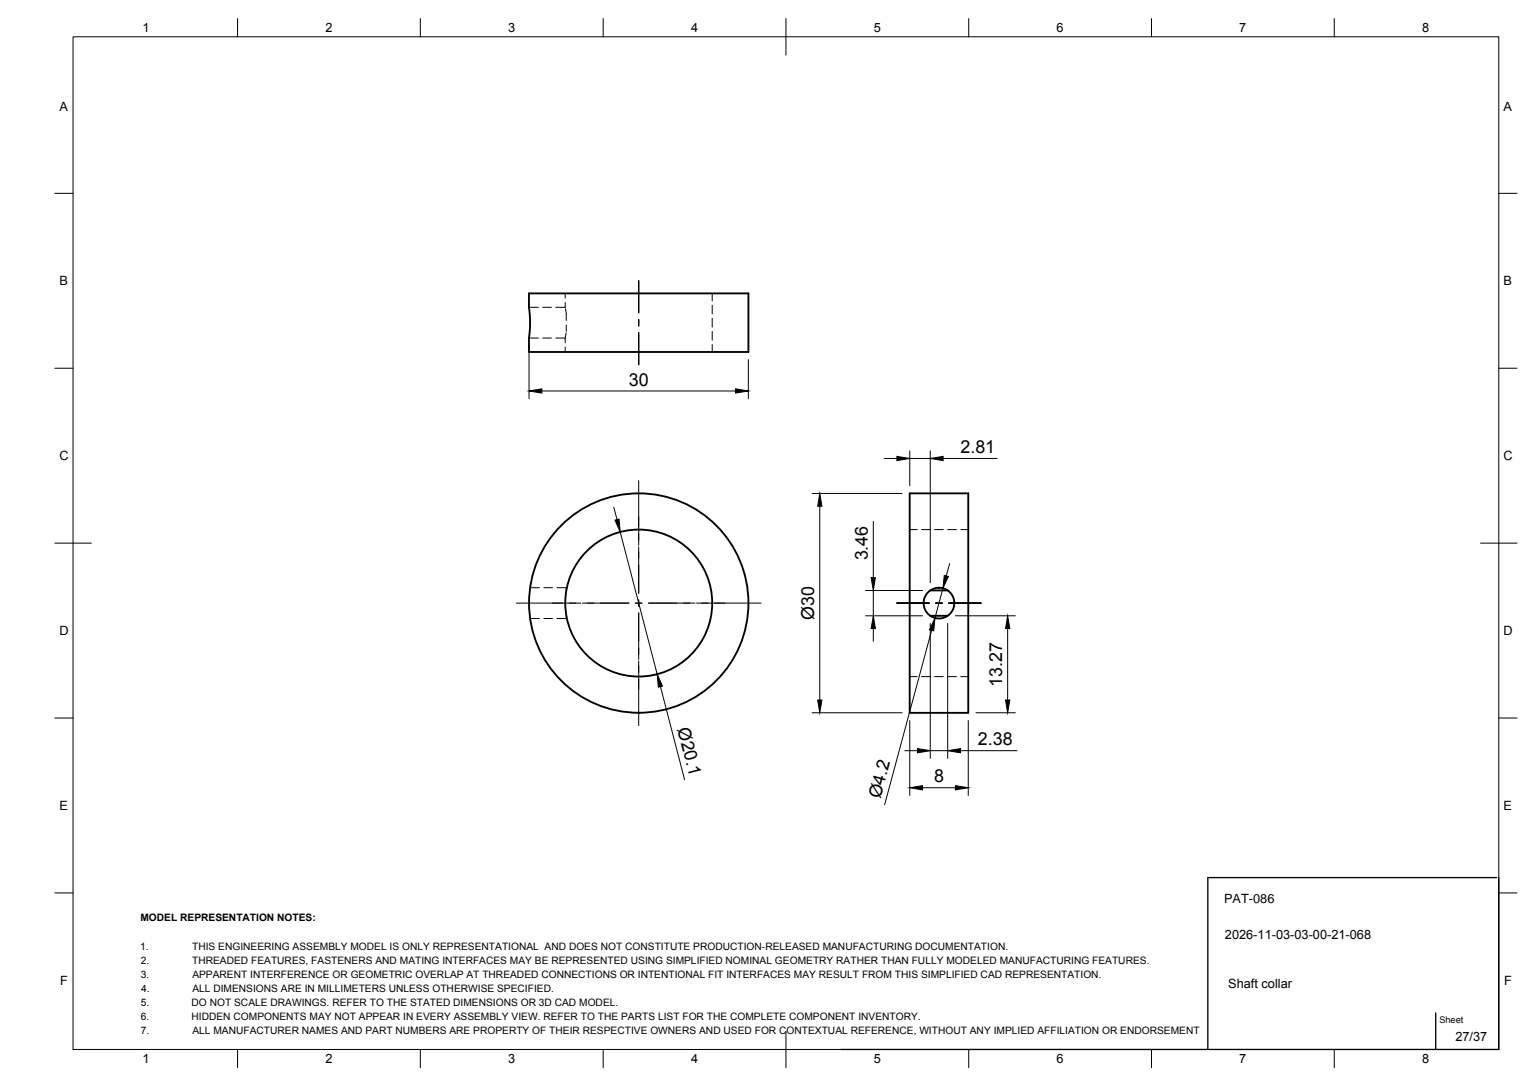
ISO-10303-21;
HEADER;
/* Generated by software containing ST-Developer
 * from STEP Tools, Inc. (www.steptools.com) 
 */

FILE_DESCRIPTION(
/* description */ ('Ratchet and pawl hand winch drum'),
/* implementation_level */ '2;1');

FILE_NAME(
/* name */ 'Shaft collar.step',
/* time_stamp */ '2026-10-27T12:42:58-07:00',
/* author */ (''),
/* organization */ (''),
/* preprocessor_version */ 'ST-DEVELOPER v20.2',
/* originating_system */ 'Autodesk Translation Framework v15.17.0.0',
/* authorisation */ '');

FILE_SCHEMA (('AUTOMOTIVE_DESIGN { 1 0 10303 214 3 1 1 }'));
ENDSEC;

DATA;
#10=MECHANICAL_DESIGN_GEOMETRIC_PRESENTATION_REPRESENTATION('',(#411),#11801);
#297=B_SPLINE_CURVE_WITH_KNOTS('',3,(#10598,#10599,#10600,#10601,#10602,
#10603,#10604,#10605,#10606,#10607,#10608,#10609,#10610,#10611),
 .UNSPECIFIED.,.F.,.F.,(4,2,2,2,2,2,4),(0.75600573798702,0.793568827564647,
0.872922520054201,0.952276212543756,1.03162990503331,1.11098359752287,1.14854668710049),
 .UNSPECIFIED.);
#298=B_SPLINE_CURVE_WITH_KNOTS('',3,(#10617,#10618,#10619,#10620,#10621,
#10622,#10623,#10624,#10625,#10626,#10627,#10628,#10629,#10630,#10631,#10632,
#10633,#10634),.UNSPECIFIED.,.F.,.F.,(4,2,2,2,2,2,2,2,4),(0.,0.079216580773363,
0.158433161546726,0.23764869707457,0.316864232602414,0.396079768130259,
0.475295303658103,0.554511884431466,0.633728465204829),.UNSPECIFIED.);
#299=B_SPLINE_CURVE_WITH_KNOTS('',3,(#10635,#10636,#10637,#10638,#10639,
#10640,#10641,#10642,#10643,#10644,#10645,#10646,#10647,#10648,#10649,#10650,
#10651,#10652),.UNSPECIFIED.,.F.,.F.,(4,2,2,2,2,2,2,2,4),(0.633728465204829,
0.712945045978192,0.792161626751555,0.871377162279399,0.950592697807243,
1.02980823333509,1.10902376886293,1.18824034963629,1.26745693040966),
 .UNSPECIFIED.);
#300=B_SPLINE_CURVE_WITH_KNOTS('',3,(#10655,#10656,#10657,#10658,#10659,
#10660,#10661,#10662,#10663,#10664,#10665,#10666,#10667,#10668),
 .UNSPECIFIED.,.F.,.F.,(4,2,2,2,2,2,4),(0.121154929624515,0.158718019202143,
0.238071711691697,0.317425404181252,0.396779096670807,0.476132789160362,
0.513695878737989),.UNSPECIFIED.);
#342=SHAPE_REPRESENTATION_RELATIONSHIP('SRR','None',#11970,#376);
#376=ADVANCED_BREP_SHAPE_REPRESENTATION('',(#444),#11787);
#411=STYLED_ITEM('',(#12213),#444);
#444=MANIFOLD_SOLID_BREP('Body1',#6290);
#564=FACE_BOUND('',#1514,.T.);
#565=FACE_BOUND('',#1516,.T.);
#566=FACE_BOUND('',#1518,.T.);
#567=FACE_BOUND('',#1520,.T.);
#728=PLANE('',#7057);
#729=PLANE('',#7062);
#730=PLANE('',#7069);
#731=PLANE('',#7070);
#1046=FACE_OUTER_BOUND('',#1510,.T.);
#1047=FACE_OUTER_BOUND('',#1511,.T.);
#1048=FACE_OUTER_BOUND('',#1512,.T.);
#1049=FACE_OUTER_BOUND('',#1513,.T.);
#1050=FACE_OUTER_BOUND('',#1515,.T.);
#1051=FACE_OUTER_BOUND('',#1517,.T.);
#1052=FACE_OUTER_BOUND('',#1519,.T.);
#1510=EDGE_LOOP('',(#5107,#5108));
#1511=EDGE_LOOP('',(#5109,#5110,#5111,#5112,#5113,#5114,#5115,#5116,#5117));
#1512=EDGE_LOOP('',(#5118,#5119,#5120));
#1513=EDGE_LOOP('',(#5121,#5122,#5123,#5124));
#1514=EDGE_LOOP('',(#5125,#5126,#5127,#5128));
#1515=EDGE_LOOP('',(#5129,#5130,#5131,#5132));
#1516=EDGE_LOOP('',(#5133,#5134));
#1517=EDGE_LOOP('',(#5135));
#1518=EDGE_LOOP('',(#5136));
#1519=EDGE_LOOP('',(#5137));
#1520=EDGE_LOOP('',(#5138));
#1959=LINE('',#10594,#2470);
#1960=LINE('',#10615,#2471);
#1961=LINE('',#10670,#2472);
#1962=LINE('',#10675,#2473);
#1963=LINE('',#10681,#2474);
#2470=VECTOR('',#8378,1.);
#2471=VECTOR('',#8385,0.21);
#2472=VECTOR('',#8390,1.);
#2473=VECTOR('',#8395,1.005);
#2474=VECTOR('',#8402,1.5);
#2863=CIRCLE('',#7058,0.21);
#2864=CIRCLE('',#7060,0.21);
#2865=CIRCLE('',#7061,0.21);
#2866=CIRCLE('',#7064,1.005);
#2867=CIRCLE('',#7065,1.005);
#2868=CIRCLE('',#7067,1.5);
#2869=CIRCLE('',#7068,1.5);
#3234=VERTEX_POINT('',#10592);
#3235=VERTEX_POINT('',#10593);
#3236=VERTEX_POINT('',#10597);
#3237=VERTEX_POINT('',#10612);
#3238=VERTEX_POINT('',#10614);
#3239=VERTEX_POINT('',#10616);
#3240=VERTEX_POINT('',#10653);
#3241=VERTEX_POINT('',#10672);
#3242=VERTEX_POINT('',#10674);
#3243=VERTEX_POINT('',#10678);
#3244=VERTEX_POINT('',#10680);
#3897=EDGE_CURVE('',#3234,#3235,#1959,.T.);
#3898=EDGE_CURVE('',#3234,#3235,#2863,.T.);
#3899=EDGE_CURVE('',#3236,#3234,#297,.T.);
#3900=EDGE_CURVE('',#3237,#3236,#2864,.T.);
#3901=EDGE_CURVE('',#3237,#3238,#1960,.T.);
#3902=EDGE_CURVE('',#3239,#3238,#298,.T.);
#3903=EDGE_CURVE('',#3238,#3239,#299,.T.);
#3904=EDGE_CURVE('',#3240,#3237,#2865,.T.);
#3905=EDGE_CURVE('',#3235,#3240,#300,.T.);
#3906=EDGE_CURVE('',#3240,#3236,#1961,.T.);
#3907=EDGE_CURVE('',#3241,#3241,#2866,.T.);
#3908=EDGE_CURVE('',#3241,#3242,#1962,.T.);
#3909=EDGE_CURVE('',#3242,#3242,#2867,.T.);
#3910=EDGE_CURVE('',#3243,#3243,#2868,.T.);
#3911=EDGE_CURVE('',#3243,#3244,#1963,.T.);
#3912=EDGE_CURVE('',#3244,#3244,#2869,.T.);
#5107=ORIENTED_EDGE('',*,*,#3897,.F.);
#5108=ORIENTED_EDGE('',*,*,#3898,.T.);
#5109=ORIENTED_EDGE('',*,*,#3899,.F.);
#5110=ORIENTED_EDGE('',*,*,#3900,.F.);
#5111=ORIENTED_EDGE('',*,*,#3901,.T.);
#5112=ORIENTED_EDGE('',*,*,#3902,.F.);
#5113=ORIENTED_EDGE('',*,*,#3903,.F.);
#5114=ORIENTED_EDGE('',*,*,#3901,.F.);
#5115=ORIENTED_EDGE('',*,*,#3904,.F.);
#5116=ORIENTED_EDGE('',*,*,#3905,.F.);
#5117=ORIENTED_EDGE('',*,*,#3898,.F.);
#5118=ORIENTED_EDGE('',*,*,#3906,.F.);
#5119=ORIENTED_EDGE('',*,*,#3904,.T.);
#5120=ORIENTED_EDGE('',*,*,#3900,.T.);
#5121=ORIENTED_EDGE('',*,*,#3907,.F.);
#5122=ORIENTED_EDGE('',*,*,#3908,.T.);
#5123=ORIENTED_EDGE('',*,*,#3909,.T.);
#5124=ORIENTED_EDGE('',*,*,#3908,.F.);
#5125=ORIENTED_EDGE('',*,*,#3905,.T.);
#5126=ORIENTED_EDGE('',*,*,#3906,.T.);
#5127=ORIENTED_EDGE('',*,*,#3899,.T.);
#5128=ORIENTED_EDGE('',*,*,#3897,.T.);
#5129=ORIENTED_EDGE('',*,*,#3910,.F.);
#5130=ORIENTED_EDGE('',*,*,#3911,.T.);
#5131=ORIENTED_EDGE('',*,*,#3912,.T.);
#5132=ORIENTED_EDGE('',*,*,#3911,.F.);
#5133=ORIENTED_EDGE('',*,*,#3902,.T.);
#5134=ORIENTED_EDGE('',*,*,#3903,.T.);
#5135=ORIENTED_EDGE('',*,*,#3910,.T.);
#5136=ORIENTED_EDGE('',*,*,#3907,.T.);
#5137=ORIENTED_EDGE('',*,*,#3912,.F.);
#5138=ORIENTED_EDGE('',*,*,#3909,.F.);
#5878=CYLINDRICAL_SURFACE('',#7059,0.21);
#5879=CYLINDRICAL_SURFACE('',#7063,1.005);
#5880=CYLINDRICAL_SURFACE('',#7066,1.5);
#6116=ADVANCED_FACE('',(#1046),#728,.T.);
#6117=ADVANCED_FACE('',(#1047),#5878,.F.);
#6118=ADVANCED_FACE('',(#1048),#729,.T.);
#6119=ADVANCED_FACE('',(#1049,#564),#5879,.F.);
#6120=ADVANCED_FACE('',(#1050,#565),#5880,.T.);
#6121=ADVANCED_FACE('',(#1051,#566),#730,.T.);
#6122=ADVANCED_FACE('',(#1052,#567),#731,.F.);
#6290=CLOSED_SHELL('',(#6116,#6117,#6118,#6119,#6120,#6121,#6122));
#7056=AXIS2_PLACEMENT_3D('',#10590,#8374,#8375);
#7057=AXIS2_PLACEMENT_3D('',#10591,#8376,#8377);
#7058=AXIS2_PLACEMENT_3D('',#10595,#8379,#8380);
#7059=AXIS2_PLACEMENT_3D('',#10596,#8381,#8382);
#7060=AXIS2_PLACEMENT_3D('',#10613,#8383,#8384);
#7061=AXIS2_PLACEMENT_3D('',#10654,#8386,#8387);
#7062=AXIS2_PLACEMENT_3D('',#10669,#8388,#8389);
#7063=AXIS2_PLACEMENT_3D('',#10671,#8391,#8392);
#7064=AXIS2_PLACEMENT_3D('',#10673,#8393,#8394);
#7065=AXIS2_PLACEMENT_3D('',#10676,#8396,#8397);
#7066=AXIS2_PLACEMENT_3D('',#10677,#8398,#8399);
#7067=AXIS2_PLACEMENT_3D('',#10679,#8400,#8401);
#7068=AXIS2_PLACEMENT_3D('',#10682,#8403,#8404);
#7069=AXIS2_PLACEMENT_3D('',#10683,#8405,#8406);
#7070=AXIS2_PLACEMENT_3D('',#10684,#8407,#8408);
#8374=DIRECTION('axis',(0.,0.,1.));
#8375=DIRECTION('refdir',(1.,0.,0.));
#8376=DIRECTION('center_axis',(0.,0.,1.));
#8377=DIRECTION('ref_axis',(1.,0.,0.));
#8378=DIRECTION('',(0.,1.,0.));
#8379=DIRECTION('center_axis',(0.,0.,1.));
#8380=DIRECTION('ref_axis',(1.,0.,0.));
#8381=DIRECTION('center_axis',(0.,0.,1.));
#8382=DIRECTION('ref_axis',(1.,0.,0.));
#8383=DIRECTION('center_axis',(0.,0.,1.));
#8384=DIRECTION('ref_axis',(1.,0.,0.));
#8385=DIRECTION('',(0.,0.,1.));
#8386=DIRECTION('center_axis',(0.,0.,1.));
#8387=DIRECTION('ref_axis',(1.,0.,0.));
#8388=DIRECTION('center_axis',(0.,0.,1.));
#8389=DIRECTION('ref_axis',(1.,0.,0.));
#8390=DIRECTION('',(0.,-1.,0.));
#8391=DIRECTION('center_axis',(0.,1.,0.));
#8392=DIRECTION('ref_axis',(1.,0.,0.));
#8393=DIRECTION('center_axis',(0.,-1.,0.));
#8394=DIRECTION('ref_axis',(1.,0.,0.));
#8395=DIRECTION('',(0.,-1.,0.));
#8396=DIRECTION('center_axis',(0.,-1.,0.));
#8397=DIRECTION('ref_axis',(1.,0.,0.));
#8398=DIRECTION('center_axis',(0.,1.,0.));
#8399=DIRECTION('ref_axis',(1.,0.,0.));
#8400=DIRECTION('center_axis',(0.,1.,0.));
#8401=DIRECTION('ref_axis',(1.,0.,0.));
#8402=DIRECTION('',(0.,-1.,0.));
#8403=DIRECTION('center_axis',(0.,1.,0.));
#8404=DIRECTION('ref_axis',(1.,0.,0.));
#8405=DIRECTION('center_axis',(0.,1.,0.));
#8406=DIRECTION('ref_axis',(1.,0.,0.));
#8407=DIRECTION('center_axis',(0.,1.,0.));
#8408=DIRECTION('ref_axis',(1.,0.,0.));
#10590=CARTESIAN_POINT('',(0.,0.,0.));
#10591=CARTESIAN_POINT('Origin',(0.,-1.25,7.52));
#10592=CARTESIAN_POINT('',(0.172988438920056,-1.36905880899792,7.52));
#10593=CARTESIAN_POINT('',(0.172988438920056,-1.13094119100209,7.52));
#10594=CARTESIAN_POINT('',(0.172988438920056,-1.65,7.52));
#10595=CARTESIAN_POINT('Origin',(0.,-1.25,7.52));
#10596=CARTESIAN_POINT('Origin',(0.,-1.25,7.52));
#10597=CARTESIAN_POINT('',(-0.172988438920056,-1.36905880899792,7.52));
#10598=CARTESIAN_POINT('Ctrl Pts',(-0.172988438920056,-1.36905880899792,
7.52));
#10599=CARTESIAN_POINT('Ctrl Pts',(-0.165594865311314,-1.37980142239529,
7.52129192197638));
#10600=CARTESIAN_POINT('Ctrl Pts',(-0.157297138725606,-1.38968770937274,
7.52265394943905));
#10601=CARTESIAN_POINT('Ctrl Pts',(-0.129892073845076,-1.41709277425327,
7.5267480843909));
#10602=CARTESIAN_POINT('Ctrl Pts',(-0.106330167759284,-1.43324205633295,
7.52969589327638));
#10603=CARTESIAN_POINT('Ctrl Pts',(-0.0546129046324105,-1.45469779396491,
7.53385029472357));
#10604=CARTESIAN_POINT('Ctrl Pts',(-0.0264512308298517,-1.46,7.535));
#10605=CARTESIAN_POINT('Ctrl Pts',(0.0264512308298516,-1.46,7.535));
#10606=CARTESIAN_POINT('Ctrl Pts',(0.0546129046324104,-1.45469779396491,
7.53385029472357));
#10607=CARTESIAN_POINT('Ctrl Pts',(0.106330167759284,-1.43324205633295,
7.52969589327638));
#10608=CARTESIAN_POINT('Ctrl Pts',(0.129892073845076,-1.41709277425327,
7.5267480843909));
#10609=CARTESIAN_POINT('Ctrl Pts',(0.157297138725606,-1.38968770937274,
7.52265394943905));
#10610=CARTESIAN_POINT('Ctrl Pts',(0.165594865311315,-1.37980142239529,
7.52129192197638));
#10611=CARTESIAN_POINT('Ctrl Pts',(0.172988438920056,-1.36905880899792,
7.52));
#10612=CARTESIAN_POINT('',(-0.21,-1.25,7.52));
#10613=CARTESIAN_POINT('Origin',(0.,-1.25,7.52));
#10614=CARTESIAN_POINT('',(-0.21,-1.25,8.01522725533839));
#10615=CARTESIAN_POINT('',(-0.21,-1.25,7.52));
#10616=CARTESIAN_POINT('',(0.21,-1.25,8.01522725533839));
#10617=CARTESIAN_POINT('Ctrl Pts',(0.21,-1.25,8.01522725533839));
#10618=CARTESIAN_POINT('Ctrl Pts',(0.21,-1.27640552692445,8.01522725533839));
#10619=CARTESIAN_POINT('Ctrl Pts',(0.204715737269596,-1.30454707409071,
8.01600415954412));
#10620=CARTESIAN_POINT('Ctrl Pts',(0.183273763036332,-1.35627626890513,
8.01880073282317));
#10621=CARTESIAN_POINT('Ctrl Pts',(0.167117923970394,-1.37986692412796,
8.02077897157582));
#10622=CARTESIAN_POINT('Ctrl Pts',(0.129867169887369,-1.41711767821098,
8.02448481141327));
#10623=CARTESIAN_POINT('Ctrl Pts',(0.106276408305765,-1.43327371000135,
8.02645455657129));
#10624=CARTESIAN_POINT('Ctrl Pts',(0.0545468514059001,-1.45471582482622,
8.02923165515645));
#10625=CARTESIAN_POINT('Ctrl Pts',(0.0264051785092814,-1.46,8.03));
#10626=CARTESIAN_POINT('Ctrl Pts',(-0.0264051785092814,-1.46,8.03));
#10627=CARTESIAN_POINT('Ctrl Pts',(-0.0545468514059,-1.45471582482622,8.02923165515645));
#10628=CARTESIAN_POINT('Ctrl Pts',(-0.106276408305765,-1.43327371000135,
8.02645455657129));
#10629=CARTESIAN_POINT('Ctrl Pts',(-0.129867169887369,-1.41711767821098,
8.02448481141327));
#10630=CARTESIAN_POINT('Ctrl Pts',(-0.167117923970394,-1.37986692412796,
8.02077897157582));
#10631=CARTESIAN_POINT('Ctrl Pts',(-0.183273763036331,-1.35627626890513,
8.01880073282317));
#10632=CARTESIAN_POINT('Ctrl Pts',(-0.204715737269596,-1.30454707409071,
8.01600415954412));
#10633=CARTESIAN_POINT('Ctrl Pts',(-0.21,-1.27640552692445,8.01522725533839));
#10634=CARTESIAN_POINT('Ctrl Pts',(-0.21,-1.25,8.01522725533839));
#10635=CARTESIAN_POINT('Ctrl Pts',(-0.21,-1.25,8.01522725533839));
#10636=CARTESIAN_POINT('Ctrl Pts',(-0.21,-1.22359447307555,8.01522725533839));
#10637=CARTESIAN_POINT('Ctrl Pts',(-0.204715737269596,-1.19545292590929,
8.01600415954412));
#10638=CARTESIAN_POINT('Ctrl Pts',(-0.183273763036332,-1.14372373109487,
8.01880073282317));
#10639=CARTESIAN_POINT('Ctrl Pts',(-0.167117923970394,-1.12013307587204,
8.02077897157582));
#10640=CARTESIAN_POINT('Ctrl Pts',(-0.129867169887369,-1.08288232178902,
8.02448481141327));
#10641=CARTESIAN_POINT('Ctrl Pts',(-0.106276408305765,-1.06672628999865,
8.02645455657129));
#10642=CARTESIAN_POINT('Ctrl Pts',(-0.0545468514059001,-1.04528417517378,
8.02923165515645));
#10643=CARTESIAN_POINT('Ctrl Pts',(-0.0264051785092814,-1.04,8.03));
#10644=CARTESIAN_POINT('Ctrl Pts',(0.0264051785092814,-1.04,8.03));
#10645=CARTESIAN_POINT('Ctrl Pts',(0.0545468514059002,-1.04528417517378,
8.02923165515645));
#10646=CARTESIAN_POINT('Ctrl Pts',(0.106276408305765,-1.06672628999865,
8.02645455657129));
#10647=CARTESIAN_POINT('Ctrl Pts',(0.129867169887369,-1.08288232178902,
8.02448481141327));
#10648=CARTESIAN_POINT('Ctrl Pts',(0.167117923970394,-1.12013307587204,
8.02077897157582));
#10649=CARTESIAN_POINT('Ctrl Pts',(0.183273763036331,-1.14372373109487,
8.01880073282317));
#10650=CARTESIAN_POINT('Ctrl Pts',(0.204715737269596,-1.19545292590929,
8.01600415954412));
#10651=CARTESIAN_POINT('Ctrl Pts',(0.21,-1.22359447307555,8.01522725533839));
#10652=CARTESIAN_POINT('Ctrl Pts',(0.21,-1.25,8.01522725533839));
#10653=CARTESIAN_POINT('',(-0.172988438920056,-1.13094119100209,7.52));
#10654=CARTESIAN_POINT('Origin',(0.,-1.25,7.52));
#10655=CARTESIAN_POINT('Ctrl Pts',(0.172988438920056,-1.13094119100209,
7.52));
#10656=CARTESIAN_POINT('Ctrl Pts',(0.165594865311315,-1.12019857760471,
7.52129192197638));
#10657=CARTESIAN_POINT('Ctrl Pts',(0.157297138725606,-1.11031229062726,
7.52265394943905));
#10658=CARTESIAN_POINT('Ctrl Pts',(0.129892073845076,-1.08290722574673,
7.5267480843909));
#10659=CARTESIAN_POINT('Ctrl Pts',(0.106330167759284,-1.06675794366705,
7.52969589327638));
#10660=CARTESIAN_POINT('Ctrl Pts',(0.0546129046324104,-1.04530220603509,
7.53385029472357));
#10661=CARTESIAN_POINT('Ctrl Pts',(0.0264512308298516,-1.04,7.535));
#10662=CARTESIAN_POINT('Ctrl Pts',(-0.0264512308298516,-1.04,7.535));
#10663=CARTESIAN_POINT('Ctrl Pts',(-0.0546129046324104,-1.04530220603509,
7.53385029472357));
#10664=CARTESIAN_POINT('Ctrl Pts',(-0.106330167759284,-1.06675794366705,
7.52969589327638));
#10665=CARTESIAN_POINT('Ctrl Pts',(-0.129892073845076,-1.08290722574673,
7.5267480843909));
#10666=CARTESIAN_POINT('Ctrl Pts',(-0.157297138725606,-1.11031229062726,
7.52265394943905));
#10667=CARTESIAN_POINT('Ctrl Pts',(-0.165594865311315,-1.12019857760471,
7.52129192197638));
#10668=CARTESIAN_POINT('Ctrl Pts',(-0.172988438920056,-1.13094119100209,
7.52));
#10669=CARTESIAN_POINT('Origin',(0.,-1.25,7.52));
#10670=CARTESIAN_POINT('',(-0.172988438920056,-1.65,7.52));
#10671=CARTESIAN_POINT('Origin',(0.,-1.65,6.53));
#10672=CARTESIAN_POINT('',(-1.005,-0.85,6.53));
#10673=CARTESIAN_POINT('Origin',(0.,-0.85,6.53));
#10674=CARTESIAN_POINT('',(-1.005,-1.65,6.53));
#10675=CARTESIAN_POINT('',(-1.005,-1.65,6.53));
#10676=CARTESIAN_POINT('Origin',(0.,-1.65,6.53));
#10677=CARTESIAN_POINT('Origin',(0.,-1.65,6.53));
#10678=CARTESIAN_POINT('',(-1.5,-0.85,6.53));
#10679=CARTESIAN_POINT('Origin',(0.,-0.85,6.53));
#10680=CARTESIAN_POINT('',(-1.5,-1.65,6.53));
#10681=CARTESIAN_POINT('',(-1.5,-1.65,6.53));
#10682=CARTESIAN_POINT('Origin',(0.,-1.65,6.53));
#10683=CARTESIAN_POINT('Origin',(0.,-0.85,6.53));
#10684=CARTESIAN_POINT('Origin',(0.,-1.65,6.53));
#11747=UNCERTAINTY_MEASURE_WITH_UNIT(LENGTH_MEASURE(0.001),#11802,
'DISTANCE_ACCURACY_VALUE',
'Maximum model space distance between geometric entities at asserted c
onnectivities');
#11761=UNCERTAINTY_MEASURE_WITH_UNIT(LENGTH_MEASURE(0.001),#11802,
'DISTANCE_ACCURACY_VALUE',
'Maximum model space distance between geometric entities at asserted c
onnectivities');
#11787=(
GEOMETRIC_REPRESENTATION_CONTEXT(3)
GLOBAL_UNCERTAINTY_ASSIGNED_CONTEXT((#11747))
GLOBAL_UNIT_ASSIGNED_CONTEXT((#11802,#11804,#11805))
REPRESENTATION_CONTEXT('','3D')
);
#11801=(
GEOMETRIC_REPRESENTATION_CONTEXT(3)
GLOBAL_UNCERTAINTY_ASSIGNED_CONTEXT((#11761))
GLOBAL_UNIT_ASSIGNED_CONTEXT((#11802,#11804,#11805))
REPRESENTATION_CONTEXT('','3D')
);
#11802=(
LENGTH_UNIT()
NAMED_UNIT(*)
SI_UNIT(.CENTI.,.METRE.)
);
#11804=(
NAMED_UNIT(*)
PLANE_ANGLE_UNIT()
SI_UNIT($,.RADIAN.)
);
#11805=(
NAMED_UNIT(*)
SI_UNIT($,.STERADIAN.)
SOLID_ANGLE_UNIT()
);
#11831=SHAPE_DEFINITION_REPRESENTATION(#11872,#11970);
#11872=PRODUCT_DEFINITION_SHAPE('',$,#12010);
#11970=SHAPE_REPRESENTATION('',(#7056),#11787);
#11984=PRODUCT_DEFINITION_CONTEXT('part definition',#12103,'design');
#12010=PRODUCT_DEFINITION('Shaft collar','Shaft collar',#12049,#11984);
#12049=PRODUCT_DEFINITION_FORMATION('',$,#12130);
#12103=APPLICATION_CONTEXT(
'Core Data for Automotive Mechanical Design Process');
#12104=PRODUCT_CONTEXT('part definition',#12103,'mechanical');
#12130=PRODUCT('Shaft collar','Shaft collar','Shaft collar',(#12104));
#12207=COLOUR_RGB('Grey',0.48,0.52,0.57);
#12208=FILL_AREA_STYLE_COLOUR('',#12207);
#12209=FILL_AREA_STYLE('',(#12208));
#12210=SURFACE_STYLE_FILL_AREA(#12209);
#12211=SURFACE_SIDE_STYLE('',(#12210));
#12212=SURFACE_STYLE_USAGE(.BOTH.,#12211);
#12213=PRESENTATION_STYLE_ASSIGNMENT((#12212));
ENDSEC;
END-ISO-10303-21;
